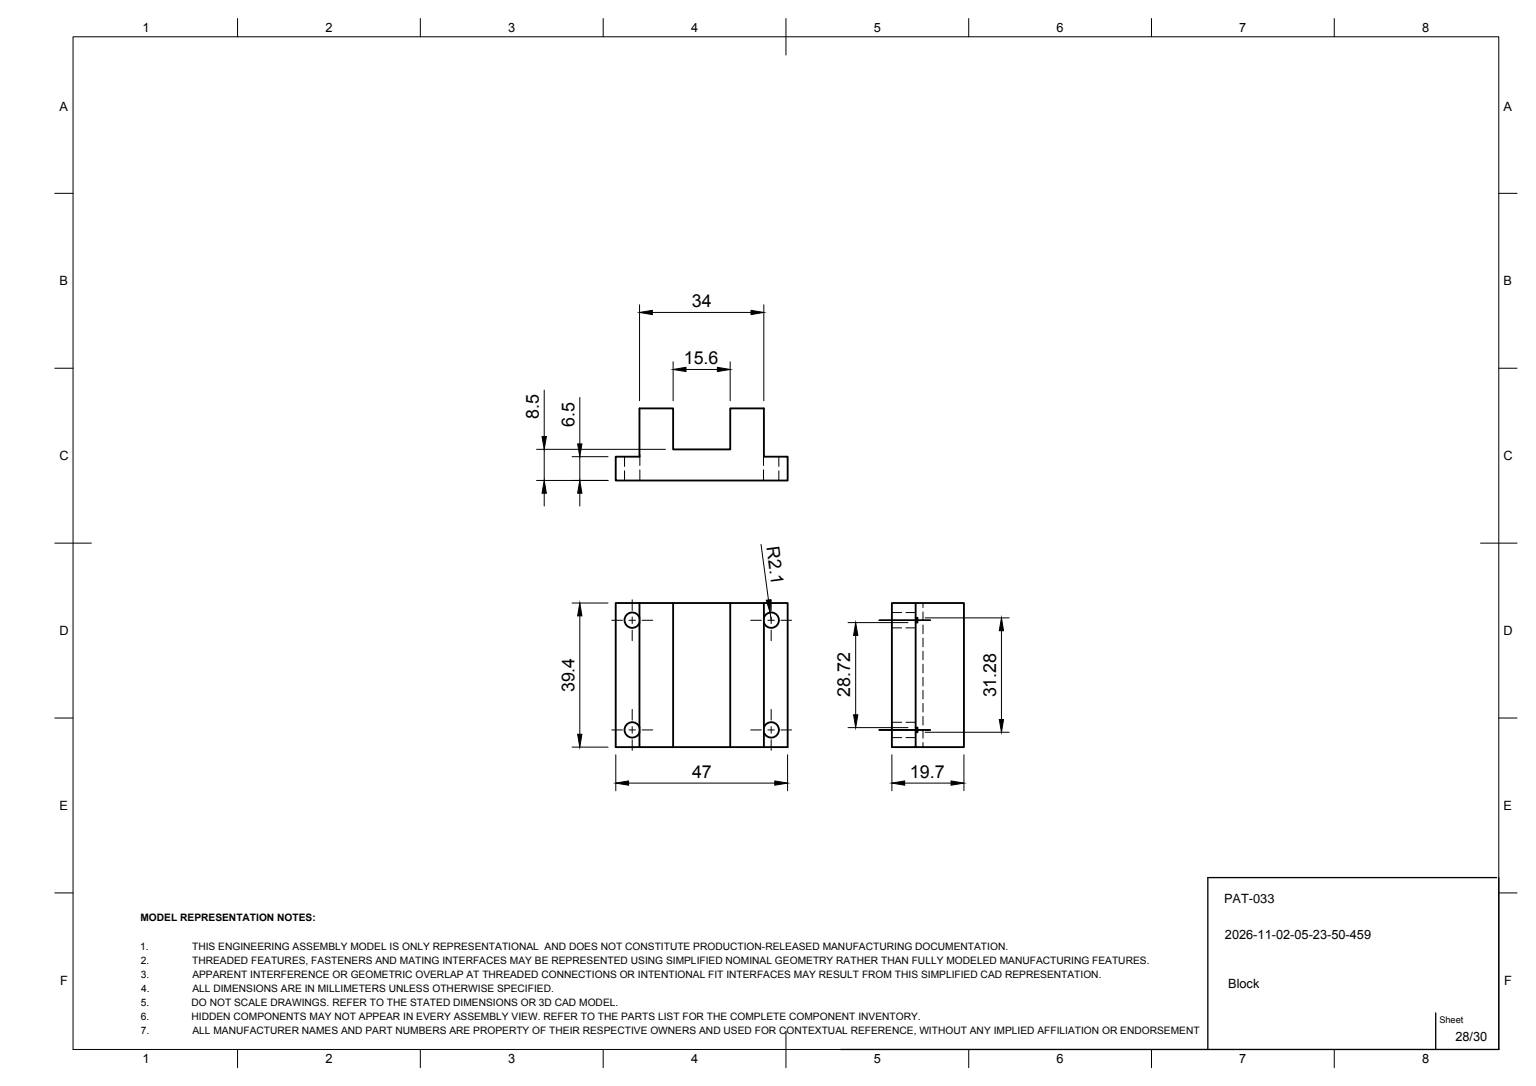
ISO-10303-21;
HEADER;
/* Generated by software containing ST-Developer
 * from STEP Tools, Inc. (www.steptools.com) 
 */

FILE_DESCRIPTION(
/* description */ ('Dual-rail gantry carriage'),
/* implementation_level */ '2;1');

FILE_NAME(
/* name */ 'Block.step',
/* time_stamp */ '2026-10-27T10:49:15-07:00',
/* author */ (''),
/* organization */ (''),
/* preprocessor_version */ 'ST-DEVELOPER v20.2',
/* originating_system */ 'Autodesk Translation Framework v15.17.0.0',
/* authorisation */ '');

FILE_SCHEMA (('AUTOMOTIVE_DESIGN { 1 0 10303 214 3 1 1 }'));
ENDSEC;

DATA;
#10=MECHANICAL_DESIGN_GEOMETRIC_PRESENTATION_REPRESENTATION('',(#607),#12804);
#545=SHAPE_REPRESENTATION_RELATIONSHIP('SRR','None',#13025,#576);
#576=ADVANCED_BREP_SHAPE_REPRESENTATION('',(#636),#12795);
#607=STYLED_ITEM('',(#13226),#636);
#636=MANIFOLD_SOLID_BREP('Body1',#7387);
#751=FACE_BOUND('',#1843,.T.);
#752=FACE_BOUND('',#1844,.T.);
#753=FACE_BOUND('',#1845,.T.);
#754=FACE_BOUND('',#1846,.T.);
#971=PLANE('',#8200);
#972=PLANE('',#8206);
#973=PLANE('',#8212);
#974=PLANE('',#8218);
#975=PLANE('',#8224);
#976=PLANE('',#8225);
#977=PLANE('',#8226);
#978=PLANE('',#8227);
#979=PLANE('',#8228);
#980=PLANE('',#8229);
#981=PLANE('',#8230);
#982=PLANE('',#8231);
#983=PLANE('',#8232);
#984=PLANE('',#8233);
#985=PLANE('',#8234);
#986=PLANE('',#8235);
#987=PLANE('',#8236);
#988=PLANE('',#8237);
#1331=FACE_OUTER_BOUND('',#1829,.T.);
#1332=FACE_OUTER_BOUND('',#1830,.T.);
#1333=FACE_OUTER_BOUND('',#1831,.T.);
#1334=FACE_OUTER_BOUND('',#1832,.T.);
#1335=FACE_OUTER_BOUND('',#1833,.T.);
#1336=FACE_OUTER_BOUND('',#1834,.T.);
#1337=FACE_OUTER_BOUND('',#1835,.T.);
#1338=FACE_OUTER_BOUND('',#1836,.T.);
#1339=FACE_OUTER_BOUND('',#1837,.T.);
#1340=FACE_OUTER_BOUND('',#1838,.T.);
#1341=FACE_OUTER_BOUND('',#1839,.T.);
#1342=FACE_OUTER_BOUND('',#1840,.T.);
#1343=FACE_OUTER_BOUND('',#1841,.T.);
#1344=FACE_OUTER_BOUND('',#1842,.T.);
#1345=FACE_OUTER_BOUND('',#1847,.T.);
#1346=FACE_OUTER_BOUND('',#1848,.T.);
#1347=FACE_OUTER_BOUND('',#1849,.T.);
#1348=FACE_OUTER_BOUND('',#1850,.T.);
#1349=FACE_OUTER_BOUND('',#1851,.T.);
#1350=FACE_OUTER_BOUND('',#1852,.T.);
#1351=FACE_OUTER_BOUND('',#1853,.T.);
#1352=FACE_OUTER_BOUND('',#1854,.T.);
#1829=EDGE_LOOP('',(#6417,#6418));
#1830=EDGE_LOOP('',(#6419,#6420,#6421,#6422,#6423,#6424,#6425,#6426));
#1831=EDGE_LOOP('',(#6427,#6428));
#1832=EDGE_LOOP('',(#6429,#6430,#6431,#6432,#6433,#6434,#6435,#6436));
#1833=EDGE_LOOP('',(#6437,#6438));
#1834=EDGE_LOOP('',(#6439,#6440,#6441,#6442,#6443,#6444,#6445,#6446));
#1835=EDGE_LOOP('',(#6447,#6448));
#1836=EDGE_LOOP('',(#6449,#6450,#6451,#6452,#6453,#6454,#6455,#6456));
#1837=EDGE_LOOP('',(#6457,#6458,#6459,#6460,#6461,#6462,#6463,#6464,#6465,
#6466,#6467,#6468));
#1838=EDGE_LOOP('',(#6469,#6470,#6471,#6472,#6473,#6474,#6475,#6476,#6477,
#6478,#6479,#6480));
#1839=EDGE_LOOP('',(#6481,#6482,#6483,#6484,#6485,#6486,#6487,#6488,#6489,
#6490,#6491,#6492));
#1840=EDGE_LOOP('',(#6493,#6494,#6495,#6496,#6497,#6498,#6499,#6500,#6501,
#6502));
#1841=EDGE_LOOP('',(#6503,#6504,#6505,#6506));
#1842=EDGE_LOOP('',(#6507,#6508,#6509,#6510));
#1843=EDGE_LOOP('',(#6511));
#1844=EDGE_LOOP('',(#6512));
#1845=EDGE_LOOP('',(#6513));
#1846=EDGE_LOOP('',(#6514));
#1847=EDGE_LOOP('',(#6515,#6516,#6517,#6518));
#1848=EDGE_LOOP('',(#6519,#6520,#6521,#6522,#6523,#6524,#6525,#6526,#6527,
#6528));
#1849=EDGE_LOOP('',(#6529,#6530,#6531,#6532));
#1850=EDGE_LOOP('',(#6533,#6534,#6535,#6536));
#1851=EDGE_LOOP('',(#6537,#6538,#6539,#6540));
#1852=EDGE_LOOP('',(#6541,#6542,#6543,#6544));
#1853=EDGE_LOOP('',(#6545,#6546,#6547,#6548));
#1854=EDGE_LOOP('',(#6549,#6550,#6551,#6552,#6553,#6554,#6555,#6556,#6557,
#6558,#6559,#6560));
#2474=LINE('',#12113,#3183);
#2475=LINE('',#12117,#3184);
#2476=LINE('',#12121,#3185);
#2477=LINE('',#12125,#3186);
#2478=LINE('',#12129,#3187);
#2479=LINE('',#12133,#3188);
#2480=LINE('',#12137,#3189);
#2481=LINE('',#12141,#3190);
#2482=LINE('',#12145,#3191);
#2483=LINE('',#12149,#3192);
#2484=LINE('',#12153,#3193);
#2485=LINE('',#12157,#3194);
#2486=LINE('',#12161,#3195);
#2487=LINE('',#12165,#3196);
#2488=LINE('',#12169,#3197);
#2489=LINE('',#12173,#3198);
#2490=LINE('',#12175,#3199);
#2491=LINE('',#12177,#3200);
#2492=LINE('',#12179,#3201);
#2493=LINE('',#12181,#3202);
#2494=LINE('',#12183,#3203);
#2495=LINE('',#12184,#3204);
#2496=LINE('',#12186,#3205);
#2497=LINE('',#12188,#3206);
#2498=LINE('',#12190,#3207);
#2499=LINE('',#12192,#3208);
#2500=LINE('',#12194,#3209);
#2501=LINE('',#12195,#3210);
#2502=LINE('',#12198,#3211);
#2503=LINE('',#12200,#3212);
#2504=LINE('',#12202,#3213);
#2505=LINE('',#12204,#3214);
#2506=LINE('',#12205,#3215);
#2507=LINE('',#12207,#3216);
#2508=LINE('',#12209,#3217);
#2509=LINE('',#12211,#3218);
#2510=LINE('',#12213,#3219);
#2511=LINE('',#12214,#3220);
#2512=LINE('',#12217,#3221);
#2513=LINE('',#12218,#3222);
#2514=LINE('',#12221,#3223);
#2515=LINE('',#12222,#3224);
#2516=LINE('',#12225,#3225);
#2517=LINE('',#12226,#3226);
#2518=LINE('',#12229,#3227);
#2519=LINE('',#12230,#3228);
#2520=LINE('',#12232,#3229);
#2521=LINE('',#12235,#3230);
#2522=LINE('',#12236,#3231);
#2523=LINE('',#12239,#3232);
#2524=LINE('',#12240,#3233);
#2525=LINE('',#12243,#3234);
#2526=LINE('',#12244,#3235);
#2527=LINE('',#12247,#3236);
#2528=LINE('',#12248,#3237);
#2529=LINE('',#12250,#3238);
#3183=VECTOR('',#9933,1.);
#3184=VECTOR('',#9938,1.);
#3185=VECTOR('',#9941,0.21);
#3186=VECTOR('',#9946,1.);
#3187=VECTOR('',#9949,1.);
#3188=VECTOR('',#9954,1.);
#3189=VECTOR('',#9957,0.21);
#3190=VECTOR('',#9962,1.);
#3191=VECTOR('',#9965,1.);
#3192=VECTOR('',#9970,1.);
#3193=VECTOR('',#9973,0.21);
#3194=VECTOR('',#9978,1.);
#3195=VECTOR('',#9981,1.);
#3196=VECTOR('',#9986,1.);
#3197=VECTOR('',#9989,0.21);
#3198=VECTOR('',#9994,1.);
#3199=VECTOR('',#9997,1.);
#3200=VECTOR('',#9998,1.);
#3201=VECTOR('',#9999,1.);
#3202=VECTOR('',#10000,1.);
#3203=VECTOR('',#10001,1.);
#3204=VECTOR('',#10002,1.);
#3205=VECTOR('',#10005,1.);
#3206=VECTOR('',#10006,1.);
#3207=VECTOR('',#10007,1.);
#3208=VECTOR('',#10008,1.);
#3209=VECTOR('',#10009,1.);
#3210=VECTOR('',#10010,1.);
#3211=VECTOR('',#10013,1.);
#3212=VECTOR('',#10014,1.);
#3213=VECTOR('',#10015,1.);
#3214=VECTOR('',#10016,1.);
#3215=VECTOR('',#10017,1.);
#3216=VECTOR('',#10018,1.);
#3217=VECTOR('',#10019,1.);
#3218=VECTOR('',#10020,1.);
#3219=VECTOR('',#10021,1.);
#3220=VECTOR('',#10022,1.);
#3221=VECTOR('',#10025,1.);
#3222=VECTOR('',#10026,1.);
#3223=VECTOR('',#10029,1.);
#3224=VECTOR('',#10030,1.);
#3225=VECTOR('',#10033,1.);
#3226=VECTOR('',#10034,1.);
#3227=VECTOR('',#10037,1.);
#3228=VECTOR('',#10038,1.);
#3229=VECTOR('',#10041,1.);
#3230=VECTOR('',#10044,1.);
#3231=VECTOR('',#10045,1.);
#3232=VECTOR('',#10048,1.);
#3233=VECTOR('',#10049,1.);
#3234=VECTOR('',#10052,1.);
#3235=VECTOR('',#10053,1.);
#3236=VECTOR('',#10056,1.);
#3237=VECTOR('',#10057,1.);
#3238=VECTOR('',#10060,1.);
#3513=CIRCLE('',#8201,0.21);
#3514=CIRCLE('',#8203,0.21);
#3515=CIRCLE('',#8204,0.21);
#3516=CIRCLE('',#8205,0.21);
#3517=CIRCLE('',#8207,0.21);
#3518=CIRCLE('',#8209,0.21);
#3519=CIRCLE('',#8210,0.21);
#3520=CIRCLE('',#8211,0.21);
#3521=CIRCLE('',#8213,0.21);
#3522=CIRCLE('',#8215,0.21);
#3523=CIRCLE('',#8216,0.21);
#3524=CIRCLE('',#8217,0.21);
#3525=CIRCLE('',#8219,0.21);
#3526=CIRCLE('',#8221,0.21);
#3527=CIRCLE('',#8222,0.21);
#3528=CIRCLE('',#8223,0.21);
#4003=VERTEX_POINT('',#12111);
#4004=VERTEX_POINT('',#12112);
#4005=VERTEX_POINT('',#12116);
#4006=VERTEX_POINT('',#12118);
#4007=VERTEX_POINT('',#12120);
#4008=VERTEX_POINT('',#12123);
#4009=VERTEX_POINT('',#12127);
#4010=VERTEX_POINT('',#12128);
#4011=VERTEX_POINT('',#12132);
#4012=VERTEX_POINT('',#12134);
#4013=VERTEX_POINT('',#12136);
#4014=VERTEX_POINT('',#12139);
#4015=VERTEX_POINT('',#12143);
#4016=VERTEX_POINT('',#12144);
#4017=VERTEX_POINT('',#12148);
#4018=VERTEX_POINT('',#12150);
#4019=VERTEX_POINT('',#12152);
#4020=VERTEX_POINT('',#12155);
#4021=VERTEX_POINT('',#12159);
#4022=VERTEX_POINT('',#12160);
#4023=VERTEX_POINT('',#12164);
#4024=VERTEX_POINT('',#12166);
#4025=VERTEX_POINT('',#12168);
#4026=VERTEX_POINT('',#12171);
#4027=VERTEX_POINT('',#12176);
#4028=VERTEX_POINT('',#12178);
#4029=VERTEX_POINT('',#12180);
#4030=VERTEX_POINT('',#12182);
#4031=VERTEX_POINT('',#12187);
#4032=VERTEX_POINT('',#12189);
#4033=VERTEX_POINT('',#12191);
#4034=VERTEX_POINT('',#12193);
#4035=VERTEX_POINT('',#12197);
#4036=VERTEX_POINT('',#12199);
#4037=VERTEX_POINT('',#12201);
#4038=VERTEX_POINT('',#12203);
#4039=VERTEX_POINT('',#12206);
#4040=VERTEX_POINT('',#12208);
#4041=VERTEX_POINT('',#12210);
#4042=VERTEX_POINT('',#12212);
#4043=VERTEX_POINT('',#12216);
#4044=VERTEX_POINT('',#12220);
#4045=VERTEX_POINT('',#12224);
#4046=VERTEX_POINT('',#12228);
#4047=VERTEX_POINT('',#12234);
#4048=VERTEX_POINT('',#12238);
#4049=VERTEX_POINT('',#12242);
#4050=VERTEX_POINT('',#12246);
#4831=EDGE_CURVE('',#4003,#4004,#2474,.T.);
#4832=EDGE_CURVE('',#4003,#4004,#3513,.T.);
#4833=EDGE_CURVE('',#4005,#4003,#2475,.T.);
#4834=EDGE_CURVE('',#4006,#4005,#3514,.T.);
#4835=EDGE_CURVE('',#4006,#4007,#2476,.T.);
#4836=EDGE_CURVE('',#4007,#4007,#3515,.T.);
#4837=EDGE_CURVE('',#4008,#4006,#3516,.T.);
#4838=EDGE_CURVE('',#4004,#4008,#2477,.T.);
#4839=EDGE_CURVE('',#4009,#4010,#2478,.T.);
#4840=EDGE_CURVE('',#4009,#4010,#3517,.T.);
#4841=EDGE_CURVE('',#4011,#4009,#2479,.T.);
#4842=EDGE_CURVE('',#4012,#4011,#3518,.T.);
#4843=EDGE_CURVE('',#4012,#4013,#2480,.T.);
#4844=EDGE_CURVE('',#4013,#4013,#3519,.T.);
#4845=EDGE_CURVE('',#4014,#4012,#3520,.T.);
#4846=EDGE_CURVE('',#4010,#4014,#2481,.T.);
#4847=EDGE_CURVE('',#4015,#4016,#2482,.T.);
#4848=EDGE_CURVE('',#4015,#4016,#3521,.T.);
#4849=EDGE_CURVE('',#4017,#4015,#2483,.T.);
#4850=EDGE_CURVE('',#4018,#4017,#3522,.T.);
#4851=EDGE_CURVE('',#4018,#4019,#2484,.T.);
#4852=EDGE_CURVE('',#4019,#4019,#3523,.T.);
#4853=EDGE_CURVE('',#4020,#4018,#3524,.T.);
#4854=EDGE_CURVE('',#4016,#4020,#2485,.T.);
#4855=EDGE_CURVE('',#4021,#4022,#2486,.T.);
#4856=EDGE_CURVE('',#4021,#4022,#3525,.T.);
#4857=EDGE_CURVE('',#4023,#4021,#2487,.T.);
#4858=EDGE_CURVE('',#4024,#4023,#3526,.T.);
#4859=EDGE_CURVE('',#4024,#4025,#2488,.T.);
#4860=EDGE_CURVE('',#4025,#4025,#3527,.T.);
#4861=EDGE_CURVE('',#4026,#4024,#3528,.T.);
#4862=EDGE_CURVE('',#4022,#4026,#2489,.T.);
#4863=EDGE_CURVE('',#4008,#4017,#2490,.T.);
#4864=EDGE_CURVE('',#4020,#4027,#2491,.T.);
#4865=EDGE_CURVE('',#4028,#4027,#2492,.T.);
#4866=EDGE_CURVE('',#4028,#4029,#2493,.T.);
#4867=EDGE_CURVE('',#4030,#4029,#2494,.T.);
#4868=EDGE_CURVE('',#4030,#4005,#2495,.T.);
#4869=EDGE_CURVE('',#4014,#4023,#2496,.T.);
#4870=EDGE_CURVE('',#4026,#4031,#2497,.T.);
#4871=EDGE_CURVE('',#4032,#4031,#2498,.T.);
#4872=EDGE_CURVE('',#4033,#4032,#2499,.T.);
#4873=EDGE_CURVE('',#4034,#4033,#2500,.T.);
#4874=EDGE_CURVE('',#4034,#4011,#2501,.T.);
#4875=EDGE_CURVE('',#4027,#4035,#2502,.T.);
#4876=EDGE_CURVE('',#4035,#4036,#2503,.T.);
#4877=EDGE_CURVE('',#4036,#4037,#2504,.T.);
#4878=EDGE_CURVE('',#4037,#4038,#2505,.T.);
#4879=EDGE_CURVE('',#4038,#4034,#2506,.T.);
#4880=EDGE_CURVE('',#4033,#4039,#2507,.T.);
#4881=EDGE_CURVE('',#4039,#4040,#2508,.T.);
#4882=EDGE_CURVE('',#4040,#4041,#2509,.T.);
#4883=EDGE_CURVE('',#4041,#4042,#2510,.T.);
#4884=EDGE_CURVE('',#4042,#4028,#2511,.T.);
#4885=EDGE_CURVE('',#4043,#4030,#2512,.T.);
#4886=EDGE_CURVE('',#4035,#4043,#2513,.T.);
#4887=EDGE_CURVE('',#4044,#4043,#2514,.T.);
#4888=EDGE_CURVE('',#4036,#4044,#2515,.T.);
#4889=EDGE_CURVE('',#4045,#4044,#2516,.T.);
#4890=EDGE_CURVE('',#4037,#4045,#2517,.T.);
#4891=EDGE_CURVE('',#4046,#4045,#2518,.T.);
#4892=EDGE_CURVE('',#4038,#4046,#2519,.T.);
#4893=EDGE_CURVE('',#4031,#4046,#2520,.T.);
#4894=EDGE_CURVE('',#4047,#4032,#2521,.T.);
#4895=EDGE_CURVE('',#4039,#4047,#2522,.T.);
#4896=EDGE_CURVE('',#4048,#4047,#2523,.T.);
#4897=EDGE_CURVE('',#4040,#4048,#2524,.T.);
#4898=EDGE_CURVE('',#4049,#4048,#2525,.T.);
#4899=EDGE_CURVE('',#4041,#4049,#2526,.T.);
#4900=EDGE_CURVE('',#4050,#4049,#2527,.T.);
#4901=EDGE_CURVE('',#4042,#4050,#2528,.T.);
#4902=EDGE_CURVE('',#4029,#4050,#2529,.T.);
#6417=ORIENTED_EDGE('',*,*,#4831,.F.);
#6418=ORIENTED_EDGE('',*,*,#4832,.T.);
#6419=ORIENTED_EDGE('',*,*,#4833,.F.);
#6420=ORIENTED_EDGE('',*,*,#4834,.F.);
#6421=ORIENTED_EDGE('',*,*,#4835,.T.);
#6422=ORIENTED_EDGE('',*,*,#4836,.F.);
#6423=ORIENTED_EDGE('',*,*,#4835,.F.);
#6424=ORIENTED_EDGE('',*,*,#4837,.F.);
#6425=ORIENTED_EDGE('',*,*,#4838,.F.);
#6426=ORIENTED_EDGE('',*,*,#4832,.F.);
#6427=ORIENTED_EDGE('',*,*,#4839,.F.);
#6428=ORIENTED_EDGE('',*,*,#4840,.T.);
#6429=ORIENTED_EDGE('',*,*,#4841,.F.);
#6430=ORIENTED_EDGE('',*,*,#4842,.F.);
#6431=ORIENTED_EDGE('',*,*,#4843,.T.);
#6432=ORIENTED_EDGE('',*,*,#4844,.F.);
#6433=ORIENTED_EDGE('',*,*,#4843,.F.);
#6434=ORIENTED_EDGE('',*,*,#4845,.F.);
#6435=ORIENTED_EDGE('',*,*,#4846,.F.);
#6436=ORIENTED_EDGE('',*,*,#4840,.F.);
#6437=ORIENTED_EDGE('',*,*,#4847,.F.);
#6438=ORIENTED_EDGE('',*,*,#4848,.T.);
#6439=ORIENTED_EDGE('',*,*,#4849,.F.);
#6440=ORIENTED_EDGE('',*,*,#4850,.F.);
#6441=ORIENTED_EDGE('',*,*,#4851,.T.);
#6442=ORIENTED_EDGE('',*,*,#4852,.F.);
#6443=ORIENTED_EDGE('',*,*,#4851,.F.);
#6444=ORIENTED_EDGE('',*,*,#4853,.F.);
#6445=ORIENTED_EDGE('',*,*,#4854,.F.);
#6446=ORIENTED_EDGE('',*,*,#4848,.F.);
#6447=ORIENTED_EDGE('',*,*,#4855,.F.);
#6448=ORIENTED_EDGE('',*,*,#4856,.T.);
#6449=ORIENTED_EDGE('',*,*,#4857,.F.);
#6450=ORIENTED_EDGE('',*,*,#4858,.F.);
#6451=ORIENTED_EDGE('',*,*,#4859,.T.);
#6452=ORIENTED_EDGE('',*,*,#4860,.F.);
#6453=ORIENTED_EDGE('',*,*,#4859,.F.);
#6454=ORIENTED_EDGE('',*,*,#4861,.F.);
#6455=ORIENTED_EDGE('',*,*,#4862,.F.);
#6456=ORIENTED_EDGE('',*,*,#4856,.F.);
#6457=ORIENTED_EDGE('',*,*,#4833,.T.);
#6458=ORIENTED_EDGE('',*,*,#4831,.T.);
#6459=ORIENTED_EDGE('',*,*,#4838,.T.);
#6460=ORIENTED_EDGE('',*,*,#4863,.T.);
#6461=ORIENTED_EDGE('',*,*,#4849,.T.);
#6462=ORIENTED_EDGE('',*,*,#4847,.T.);
#6463=ORIENTED_EDGE('',*,*,#4854,.T.);
#6464=ORIENTED_EDGE('',*,*,#4864,.T.);
#6465=ORIENTED_EDGE('',*,*,#4865,.F.);
#6466=ORIENTED_EDGE('',*,*,#4866,.T.);
#6467=ORIENTED_EDGE('',*,*,#4867,.F.);
#6468=ORIENTED_EDGE('',*,*,#4868,.T.);
#6469=ORIENTED_EDGE('',*,*,#4841,.T.);
#6470=ORIENTED_EDGE('',*,*,#4839,.T.);
#6471=ORIENTED_EDGE('',*,*,#4846,.T.);
#6472=ORIENTED_EDGE('',*,*,#4869,.T.);
#6473=ORIENTED_EDGE('',*,*,#4857,.T.);
#6474=ORIENTED_EDGE('',*,*,#4855,.T.);
#6475=ORIENTED_EDGE('',*,*,#4862,.T.);
#6476=ORIENTED_EDGE('',*,*,#4870,.T.);
#6477=ORIENTED_EDGE('',*,*,#4871,.F.);
#6478=ORIENTED_EDGE('',*,*,#4872,.F.);
#6479=ORIENTED_EDGE('',*,*,#4873,.F.);
#6480=ORIENTED_EDGE('',*,*,#4874,.T.);
#6481=ORIENTED_EDGE('',*,*,#4865,.T.);
#6482=ORIENTED_EDGE('',*,*,#4875,.T.);
#6483=ORIENTED_EDGE('',*,*,#4876,.T.);
#6484=ORIENTED_EDGE('',*,*,#4877,.T.);
#6485=ORIENTED_EDGE('',*,*,#4878,.T.);
#6486=ORIENTED_EDGE('',*,*,#4879,.T.);
#6487=ORIENTED_EDGE('',*,*,#4873,.T.);
#6488=ORIENTED_EDGE('',*,*,#4880,.T.);
#6489=ORIENTED_EDGE('',*,*,#4881,.T.);
#6490=ORIENTED_EDGE('',*,*,#4882,.T.);
#6491=ORIENTED_EDGE('',*,*,#4883,.T.);
#6492=ORIENTED_EDGE('',*,*,#4884,.T.);
#6493=ORIENTED_EDGE('',*,*,#4837,.T.);
#6494=ORIENTED_EDGE('',*,*,#4834,.T.);
#6495=ORIENTED_EDGE('',*,*,#4868,.F.);
#6496=ORIENTED_EDGE('',*,*,#4885,.F.);
#6497=ORIENTED_EDGE('',*,*,#4886,.F.);
#6498=ORIENTED_EDGE('',*,*,#4875,.F.);
#6499=ORIENTED_EDGE('',*,*,#4864,.F.);
#6500=ORIENTED_EDGE('',*,*,#4853,.T.);
#6501=ORIENTED_EDGE('',*,*,#4850,.T.);
#6502=ORIENTED_EDGE('',*,*,#4863,.F.);
#6503=ORIENTED_EDGE('',*,*,#4886,.T.);
#6504=ORIENTED_EDGE('',*,*,#4887,.F.);
#6505=ORIENTED_EDGE('',*,*,#4888,.F.);
#6506=ORIENTED_EDGE('',*,*,#4876,.F.);
#6507=ORIENTED_EDGE('',*,*,#4888,.T.);
#6508=ORIENTED_EDGE('',*,*,#4889,.F.);
#6509=ORIENTED_EDGE('',*,*,#4890,.F.);
#6510=ORIENTED_EDGE('',*,*,#4877,.F.);
#6511=ORIENTED_EDGE('',*,*,#4836,.T.);
#6512=ORIENTED_EDGE('',*,*,#4844,.T.);
#6513=ORIENTED_EDGE('',*,*,#4852,.T.);
#6514=ORIENTED_EDGE('',*,*,#4860,.T.);
#6515=ORIENTED_EDGE('',*,*,#4890,.T.);
#6516=ORIENTED_EDGE('',*,*,#4891,.F.);
#6517=ORIENTED_EDGE('',*,*,#4892,.F.);
#6518=ORIENTED_EDGE('',*,*,#4878,.F.);
#6519=ORIENTED_EDGE('',*,*,#4845,.T.);
#6520=ORIENTED_EDGE('',*,*,#4842,.T.);
#6521=ORIENTED_EDGE('',*,*,#4874,.F.);
#6522=ORIENTED_EDGE('',*,*,#4879,.F.);
#6523=ORIENTED_EDGE('',*,*,#4892,.T.);
#6524=ORIENTED_EDGE('',*,*,#4893,.F.);
#6525=ORIENTED_EDGE('',*,*,#4870,.F.);
#6526=ORIENTED_EDGE('',*,*,#4861,.T.);
#6527=ORIENTED_EDGE('',*,*,#4858,.T.);
#6528=ORIENTED_EDGE('',*,*,#4869,.F.);
#6529=ORIENTED_EDGE('',*,*,#4872,.T.);
#6530=ORIENTED_EDGE('',*,*,#4894,.F.);
#6531=ORIENTED_EDGE('',*,*,#4895,.F.);
#6532=ORIENTED_EDGE('',*,*,#4880,.F.);
#6533=ORIENTED_EDGE('',*,*,#4895,.T.);
#6534=ORIENTED_EDGE('',*,*,#4896,.F.);
#6535=ORIENTED_EDGE('',*,*,#4897,.F.);
#6536=ORIENTED_EDGE('',*,*,#4881,.F.);
#6537=ORIENTED_EDGE('',*,*,#4897,.T.);
#6538=ORIENTED_EDGE('',*,*,#4898,.F.);
#6539=ORIENTED_EDGE('',*,*,#4899,.F.);
#6540=ORIENTED_EDGE('',*,*,#4882,.F.);
#6541=ORIENTED_EDGE('',*,*,#4899,.T.);
#6542=ORIENTED_EDGE('',*,*,#4900,.F.);
#6543=ORIENTED_EDGE('',*,*,#4901,.F.);
#6544=ORIENTED_EDGE('',*,*,#4883,.F.);
#6545=ORIENTED_EDGE('',*,*,#4901,.T.);
#6546=ORIENTED_EDGE('',*,*,#4902,.F.);
#6547=ORIENTED_EDGE('',*,*,#4866,.F.);
#6548=ORIENTED_EDGE('',*,*,#4884,.F.);
#6549=ORIENTED_EDGE('',*,*,#4867,.T.);
#6550=ORIENTED_EDGE('',*,*,#4902,.T.);
#6551=ORIENTED_EDGE('',*,*,#4900,.T.);
#6552=ORIENTED_EDGE('',*,*,#4898,.T.);
#6553=ORIENTED_EDGE('',*,*,#4896,.T.);
#6554=ORIENTED_EDGE('',*,*,#4894,.T.);
#6555=ORIENTED_EDGE('',*,*,#4871,.T.);
#6556=ORIENTED_EDGE('',*,*,#4893,.T.);
#6557=ORIENTED_EDGE('',*,*,#4891,.T.);
#6558=ORIENTED_EDGE('',*,*,#4889,.T.);
#6559=ORIENTED_EDGE('',*,*,#4887,.T.);
#6560=ORIENTED_EDGE('',*,*,#4885,.T.);
#6958=CYLINDRICAL_SURFACE('',#8202,0.21);
#6959=CYLINDRICAL_SURFACE('',#8208,0.21);
#6960=CYLINDRICAL_SURFACE('',#8214,0.21);
#6961=CYLINDRICAL_SURFACE('',#8220,0.21);
#7257=ADVANCED_FACE('',(#1331),#971,.T.);
#7258=ADVANCED_FACE('',(#1332),#6958,.F.);
#7259=ADVANCED_FACE('',(#1333),#972,.T.);
#7260=ADVANCED_FACE('',(#1334),#6959,.F.);
#7261=ADVANCED_FACE('',(#1335),#973,.T.);
#7262=ADVANCED_FACE('',(#1336),#6960,.F.);
#7263=ADVANCED_FACE('',(#1337),#974,.T.);
#7264=ADVANCED_FACE('',(#1338),#6961,.F.);
#7265=ADVANCED_FACE('',(#1339),#975,.T.);
#7266=ADVANCED_FACE('',(#1340),#976,.T.);
#7267=ADVANCED_FACE('',(#1341),#977,.T.);
#7268=ADVANCED_FACE('',(#1342),#978,.T.);
#7269=ADVANCED_FACE('',(#1343),#979,.T.);
#7270=ADVANCED_FACE('',(#1344,#751,#752,#753,#754),#980,.T.);
#7271=ADVANCED_FACE('',(#1345),#981,.T.);
#7272=ADVANCED_FACE('',(#1346),#982,.T.);
#7273=ADVANCED_FACE('',(#1347),#983,.T.);
#7274=ADVANCED_FACE('',(#1348),#984,.T.);
#7275=ADVANCED_FACE('',(#1349),#985,.T.);
#7276=ADVANCED_FACE('',(#1350),#986,.T.);
#7277=ADVANCED_FACE('',(#1351),#987,.T.);
#7278=ADVANCED_FACE('',(#1352),#988,.T.);
#7387=CLOSED_SHELL('',(#7257,#7258,#7259,#7260,#7261,#7262,#7263,#7264,
#7265,#7266,#7267,#7268,#7269,#7270,#7271,#7272,#7273,#7274,#7275,#7276,
#7277,#7278));
#8199=AXIS2_PLACEMENT_3D('',#12109,#9929,#9930);
#8200=AXIS2_PLACEMENT_3D('',#12110,#9931,#9932);
#8201=AXIS2_PLACEMENT_3D('',#12114,#9934,#9935);
#8202=AXIS2_PLACEMENT_3D('',#12115,#9936,#9937);
#8203=AXIS2_PLACEMENT_3D('',#12119,#9939,#9940);
#8204=AXIS2_PLACEMENT_3D('',#12122,#9942,#9943);
#8205=AXIS2_PLACEMENT_3D('',#12124,#9944,#9945);
#8206=AXIS2_PLACEMENT_3D('',#12126,#9947,#9948);
#8207=AXIS2_PLACEMENT_3D('',#12130,#9950,#9951);
#8208=AXIS2_PLACEMENT_3D('',#12131,#9952,#9953);
#8209=AXIS2_PLACEMENT_3D('',#12135,#9955,#9956);
#8210=AXIS2_PLACEMENT_3D('',#12138,#9958,#9959);
#8211=AXIS2_PLACEMENT_3D('',#12140,#9960,#9961);
#8212=AXIS2_PLACEMENT_3D('',#12142,#9963,#9964);
#8213=AXIS2_PLACEMENT_3D('',#12146,#9966,#9967);
#8214=AXIS2_PLACEMENT_3D('',#12147,#9968,#9969);
#8215=AXIS2_PLACEMENT_3D('',#12151,#9971,#9972);
#8216=AXIS2_PLACEMENT_3D('',#12154,#9974,#9975);
#8217=AXIS2_PLACEMENT_3D('',#12156,#9976,#9977);
#8218=AXIS2_PLACEMENT_3D('',#12158,#9979,#9980);
#8219=AXIS2_PLACEMENT_3D('',#12162,#9982,#9983);
#8220=AXIS2_PLACEMENT_3D('',#12163,#9984,#9985);
#8221=AXIS2_PLACEMENT_3D('',#12167,#9987,#9988);
#8222=AXIS2_PLACEMENT_3D('',#12170,#9990,#9991);
#8223=AXIS2_PLACEMENT_3D('',#12172,#9992,#9993);
#8224=AXIS2_PLACEMENT_3D('',#12174,#9995,#9996);
#8225=AXIS2_PLACEMENT_3D('',#12185,#10003,#10004);
#8226=AXIS2_PLACEMENT_3D('',#12196,#10011,#10012);
#8227=AXIS2_PLACEMENT_3D('',#12215,#10023,#10024);
#8228=AXIS2_PLACEMENT_3D('',#12219,#10027,#10028);
#8229=AXIS2_PLACEMENT_3D('',#12223,#10031,#10032);
#8230=AXIS2_PLACEMENT_3D('',#12227,#10035,#10036);
#8231=AXIS2_PLACEMENT_3D('',#12231,#10039,#10040);
#8232=AXIS2_PLACEMENT_3D('',#12233,#10042,#10043);
#8233=AXIS2_PLACEMENT_3D('',#12237,#10046,#10047);
#8234=AXIS2_PLACEMENT_3D('',#12241,#10050,#10051);
#8235=AXIS2_PLACEMENT_3D('',#12245,#10054,#10055);
#8236=AXIS2_PLACEMENT_3D('',#12249,#10058,#10059);
#8237=AXIS2_PLACEMENT_3D('',#12251,#10061,#10062);
#9929=DIRECTION('axis',(0.,0.,1.));
#9930=DIRECTION('refdir',(1.,0.,0.));
#9931=DIRECTION('center_axis',(0.,0.,1.));
#9932=DIRECTION('ref_axis',(1.,0.,0.));
#9933=DIRECTION('',(-1.,0.,0.));
#9934=DIRECTION('center_axis',(0.,0.,1.));
#9935=DIRECTION('ref_axis',(1.,0.,0.));
#9936=DIRECTION('center_axis',(0.,0.,1.));
#9937=DIRECTION('ref_axis',(1.,0.,0.));
#9938=DIRECTION('',(0.,0.,-1.));
#9939=DIRECTION('center_axis',(0.,0.,1.));
#9940=DIRECTION('ref_axis',(1.,0.,0.));
#9941=DIRECTION('',(0.,0.,1.));
#9942=DIRECTION('center_axis',(0.,0.,-1.));
#9943=DIRECTION('ref_axis',(1.,0.,0.));
#9944=DIRECTION('center_axis',(0.,0.,1.));
#9945=DIRECTION('ref_axis',(1.,0.,0.));
#9946=DIRECTION('',(0.,0.,1.));
#9947=DIRECTION('center_axis',(0.,0.,1.));
#9948=DIRECTION('ref_axis',(1.,0.,0.));
#9949=DIRECTION('',(1.,0.,0.));
#9950=DIRECTION('center_axis',(0.,0.,1.));
#9951=DIRECTION('ref_axis',(1.,0.,0.));
#9952=DIRECTION('center_axis',(0.,0.,1.));
#9953=DIRECTION('ref_axis',(1.,0.,0.));
#9954=DIRECTION('',(0.,0.,-1.));
#9955=DIRECTION('center_axis',(0.,0.,1.));
#9956=DIRECTION('ref_axis',(1.,0.,0.));
#9957=DIRECTION('',(0.,0.,1.));
#9958=DIRECTION('center_axis',(0.,0.,-1.));
#9959=DIRECTION('ref_axis',(1.,0.,0.));
#9960=DIRECTION('center_axis',(0.,0.,1.));
#9961=DIRECTION('ref_axis',(1.,0.,0.));
#9962=DIRECTION('',(0.,0.,1.));
#9963=DIRECTION('center_axis',(0.,0.,1.));
#9964=DIRECTION('ref_axis',(1.,0.,0.));
#9965=DIRECTION('',(-1.,0.,0.));
#9966=DIRECTION('center_axis',(0.,0.,1.));
#9967=DIRECTION('ref_axis',(1.,0.,0.));
#9968=DIRECTION('center_axis',(0.,0.,1.));
#9969=DIRECTION('ref_axis',(1.,0.,0.));
#9970=DIRECTION('',(0.,0.,-1.));
#9971=DIRECTION('center_axis',(0.,0.,1.));
#9972=DIRECTION('ref_axis',(1.,0.,0.));
#9973=DIRECTION('',(0.,0.,1.));
#9974=DIRECTION('center_axis',(0.,0.,-1.));
#9975=DIRECTION('ref_axis',(1.,0.,0.));
#9976=DIRECTION('center_axis',(0.,0.,1.));
#9977=DIRECTION('ref_axis',(1.,0.,0.));
#9978=DIRECTION('',(0.,0.,1.));
#9979=DIRECTION('center_axis',(0.,0.,1.));
#9980=DIRECTION('ref_axis',(1.,0.,0.));
#9981=DIRECTION('',(1.,0.,0.));
#9982=DIRECTION('center_axis',(0.,0.,1.));
#9983=DIRECTION('ref_axis',(1.,0.,0.));
#9984=DIRECTION('center_axis',(0.,0.,1.));
#9985=DIRECTION('ref_axis',(1.,0.,0.));
#9986=DIRECTION('',(0.,0.,-1.));
#9987=DIRECTION('center_axis',(0.,0.,1.));
#9988=DIRECTION('ref_axis',(1.,0.,0.));
#9989=DIRECTION('',(0.,0.,1.));
#9990=DIRECTION('center_axis',(0.,0.,-1.));
#9991=DIRECTION('ref_axis',(1.,0.,0.));
#9992=DIRECTION('center_axis',(0.,0.,1.));
#9993=DIRECTION('ref_axis',(1.,0.,0.));
#9994=DIRECTION('',(0.,0.,1.));
#9995=DIRECTION('center_axis',(0.,-1.,0.));
#9996=DIRECTION('ref_axis',(0.,0.,-1.));
#9997=DIRECTION('',(-1.,0.,0.));
#9998=DIRECTION('',(-1.,0.,0.));
#9999=DIRECTION('',(0.,0.,1.));
#10000=DIRECTION('',(1.,0.,0.));
#10001=DIRECTION('',(0.,0.,-1.));
#10002=DIRECTION('',(-1.,0.,0.));
#10003=DIRECTION('center_axis',(0.,1.,0.));
#10004=DIRECTION('ref_axis',(0.,0.,1.));
#10005=DIRECTION('',(1.,0.,0.));
#10006=DIRECTION('',(1.,0.,0.));
#10007=DIRECTION('',(0.,0.,1.));
#10008=DIRECTION('',(1.,0.,0.));
#10009=DIRECTION('',(0.,0.,-1.));
#10010=DIRECTION('',(1.,0.,0.));
#10011=DIRECTION('center_axis',(-1.,0.,0.));
#10012=DIRECTION('ref_axis',(0.,0.,1.));
#10013=DIRECTION('',(0.,-1.,0.));
#10014=DIRECTION('',(0.,0.,1.));
#10015=DIRECTION('',(0.,1.,0.));
#10016=DIRECTION('',(0.,0.,-1.));
#10017=DIRECTION('',(0.,-1.,0.));
#10018=DIRECTION('',(0.,-1.,0.));
#10019=DIRECTION('',(0.,0.,1.));
#10020=DIRECTION('',(0.,-1.,0.));
#10021=DIRECTION('',(0.,0.,-1.));
#10022=DIRECTION('',(0.,-1.,0.));
#10023=DIRECTION('center_axis',(0.,0.,-1.));
#10024=DIRECTION('ref_axis',(0.,1.,0.));
#10025=DIRECTION('',(0.,1.,0.));
#10026=DIRECTION('',(1.,0.,0.));
#10027=DIRECTION('center_axis',(0.,-1.,0.));
#10028=DIRECTION('ref_axis',(0.,0.,-1.));
#10029=DIRECTION('',(0.,0.,-1.));
#10030=DIRECTION('',(1.,0.,0.));
#10031=DIRECTION('center_axis',(0.,0.,1.));
#10032=DIRECTION('ref_axis',(0.,-1.,0.));
#10033=DIRECTION('',(0.,-1.,0.));
#10034=DIRECTION('',(1.,0.,0.));
#10035=DIRECTION('center_axis',(0.,1.,0.));
#10036=DIRECTION('ref_axis',(0.,0.,1.));
#10037=DIRECTION('',(0.,0.,1.));
#10038=DIRECTION('',(1.,0.,0.));
#10039=DIRECTION('center_axis',(0.,0.,-1.));
#10040=DIRECTION('ref_axis',(0.,1.,0.));
#10041=DIRECTION('',(0.,1.,0.));
#10042=DIRECTION('center_axis',(0.,0.,-1.));
#10043=DIRECTION('ref_axis',(0.,1.,0.));
#10044=DIRECTION('',(0.,1.,0.));
#10045=DIRECTION('',(1.,0.,0.));
#10046=DIRECTION('center_axis',(0.,-1.,0.));
#10047=DIRECTION('ref_axis',(0.,0.,-1.));
#10048=DIRECTION('',(0.,0.,-1.));
#10049=DIRECTION('',(1.,0.,0.));
#10050=DIRECTION('center_axis',(0.,0.,-1.));
#10051=DIRECTION('ref_axis',(0.,1.,0.));
#10052=DIRECTION('',(0.,1.,0.));
#10053=DIRECTION('',(1.,0.,0.));
#10054=DIRECTION('center_axis',(0.,1.,0.));
#10055=DIRECTION('ref_axis',(0.,0.,1.));
#10056=DIRECTION('',(0.,0.,1.));
#10057=DIRECTION('',(1.,0.,0.));
#10058=DIRECTION('center_axis',(0.,0.,-1.));
#10059=DIRECTION('ref_axis',(0.,1.,0.));
#10060=DIRECTION('',(0.,1.,0.));
#10061=DIRECTION('center_axis',(1.,0.,0.));
#10062=DIRECTION('ref_axis',(0.,0.,-1.));
#12109=CARTESIAN_POINT('',(0.,0.,0.));
#12110=CARTESIAN_POINT('Origin',(1.5,-1.9,1.7));
#12111=CARTESIAN_POINT('',(1.56403124237433,-1.7,1.7));
#12112=CARTESIAN_POINT('',(1.43596875762567,-1.7,1.7));
#12113=CARTESIAN_POINT('',(0.75,-1.7,1.7));
#12114=CARTESIAN_POINT('Origin',(1.5,-1.9,1.7));
#12115=CARTESIAN_POINT('Origin',(1.5,-1.9,1.7));
#12116=CARTESIAN_POINT('',(1.56403124237433,-1.7,1.75));
#12117=CARTESIAN_POINT('',(1.56403124237433,-1.7,1.7));
#12118=CARTESIAN_POINT('',(1.29,-1.9,1.75));
#12119=CARTESIAN_POINT('Origin',(1.5,-1.9,1.75));
#12120=CARTESIAN_POINT('',(1.29,-1.9,2.4));
#12121=CARTESIAN_POINT('',(1.29,-1.9,1.7));
#12122=CARTESIAN_POINT('Origin',(1.5,-1.9,2.4));
#12123=CARTESIAN_POINT('',(1.43596875762567,-1.7,1.75));
#12124=CARTESIAN_POINT('Origin',(1.5,-1.9,1.75));
#12125=CARTESIAN_POINT('',(1.43596875762567,-1.7,1.7));
#12126=CARTESIAN_POINT('Origin',(-1.5,1.9,1.7));
#12127=CARTESIAN_POINT('',(-1.56403124237433,1.7,1.7));
#12128=CARTESIAN_POINT('',(-1.43596875762567,1.7,1.7));
#12129=CARTESIAN_POINT('',(-0.75,1.7,1.7));
#12130=CARTESIAN_POINT('Origin',(-1.5,1.9,1.7));
#12131=CARTESIAN_POINT('Origin',(-1.5,1.9,1.7));
#12132=CARTESIAN_POINT('',(-1.56403124237433,1.7,1.75));
#12133=CARTESIAN_POINT('',(-1.56403124237433,1.7,1.7));
#12134=CARTESIAN_POINT('',(-1.71,1.9,1.75));
#12135=CARTESIAN_POINT('Origin',(-1.5,1.9,1.75));
#12136=CARTESIAN_POINT('',(-1.71,1.9,2.4));
#12137=CARTESIAN_POINT('',(-1.71,1.9,1.7));
#12138=CARTESIAN_POINT('Origin',(-1.5,1.9,2.4));
#12139=CARTESIAN_POINT('',(-1.43596875762567,1.7,1.75));
#12140=CARTESIAN_POINT('Origin',(-1.5,1.9,1.75));
#12141=CARTESIAN_POINT('',(-1.43596875762567,1.7,1.7));
#12142=CARTESIAN_POINT('Origin',(-1.5,-1.9,1.7));
#12143=CARTESIAN_POINT('',(-1.43596875762567,-1.7,1.7));
#12144=CARTESIAN_POINT('',(-1.56403124237433,-1.7,1.7));
#12145=CARTESIAN_POINT('',(-0.75,-1.7,1.7));
#12146=CARTESIAN_POINT('Origin',(-1.5,-1.9,1.7));
#12147=CARTESIAN_POINT('Origin',(-1.5,-1.9,1.7));
#12148=CARTESIAN_POINT('',(-1.43596875762567,-1.7,1.75));
#12149=CARTESIAN_POINT('',(-1.43596875762567,-1.7,1.7));
#12150=CARTESIAN_POINT('',(-1.71,-1.9,1.75));
#12151=CARTESIAN_POINT('Origin',(-1.5,-1.9,1.75));
#12152=CARTESIAN_POINT('',(-1.71,-1.9,2.4));
#12153=CARTESIAN_POINT('',(-1.71,-1.9,1.7));
#12154=CARTESIAN_POINT('Origin',(-1.5,-1.9,2.4));
#12155=CARTESIAN_POINT('',(-1.56403124237433,-1.7,1.75));
#12156=CARTESIAN_POINT('Origin',(-1.5,-1.9,1.75));
#12157=CARTESIAN_POINT('',(-1.56403124237433,-1.7,1.7));
#12158=CARTESIAN_POINT('Origin',(1.5,1.9,1.7));
#12159=CARTESIAN_POINT('',(1.43596875762567,1.7,1.7));
#12160=CARTESIAN_POINT('',(1.56403124237433,1.7,1.7));
#12161=CARTESIAN_POINT('',(0.75,1.7,1.7));
#12162=CARTESIAN_POINT('Origin',(1.5,1.9,1.7));
#12163=CARTESIAN_POINT('Origin',(1.5,1.9,1.7));
#12164=CARTESIAN_POINT('',(1.43596875762567,1.7,1.75));
#12165=CARTESIAN_POINT('',(1.43596875762567,1.7,1.7));
#12166=CARTESIAN_POINT('',(1.29,1.9,1.75));
#12167=CARTESIAN_POINT('Origin',(1.5,1.9,1.75));
#12168=CARTESIAN_POINT('',(1.29,1.9,2.4));
#12169=CARTESIAN_POINT('',(1.29,1.9,1.7));
#12170=CARTESIAN_POINT('Origin',(1.5,1.9,2.4));
#12171=CARTESIAN_POINT('',(1.56403124237433,1.7,1.75));
#12172=CARTESIAN_POINT('Origin',(1.5,1.9,1.75));
#12173=CARTESIAN_POINT('',(1.56403124237433,1.7,1.7));
#12174=CARTESIAN_POINT('Origin',(0.,-1.7,1.75));
#12175=CARTESIAN_POINT('',(0.,-1.7,1.75));
#12176=CARTESIAN_POINT('',(-1.97,-1.7,1.75));
#12177=CARTESIAN_POINT('',(0.,-1.7,1.75));
#12178=CARTESIAN_POINT('',(-1.97,-1.7,0.43));
#12179=CARTESIAN_POINT('',(-1.97,-1.7,1.75));
#12180=CARTESIAN_POINT('',(1.97,-1.7,0.43));
#12181=CARTESIAN_POINT('',(0.,-1.7,0.43));
#12182=CARTESIAN_POINT('',(1.97,-1.7,1.75));
#12183=CARTESIAN_POINT('',(1.97,-1.7,1.75));
#12184=CARTESIAN_POINT('',(0.,-1.7,1.75));
#12185=CARTESIAN_POINT('Origin',(0.,1.7,0.43));
#12186=CARTESIAN_POINT('',(0.,1.7,1.75));
#12187=CARTESIAN_POINT('',(1.97,1.7,1.75));
#12188=CARTESIAN_POINT('',(0.,1.7,1.75));
#12189=CARTESIAN_POINT('',(1.97,1.7,0.43));
#12190=CARTESIAN_POINT('',(1.97,1.7,0.43));
#12191=CARTESIAN_POINT('',(-1.97,1.7,0.43));
#12192=CARTESIAN_POINT('',(0.,1.7,0.43));
#12193=CARTESIAN_POINT('',(-1.97,1.7,1.75));
#12194=CARTESIAN_POINT('',(-1.97,1.7,0.43));
#12195=CARTESIAN_POINT('',(0.,1.7,1.75));
#12196=CARTESIAN_POINT('Origin',(-1.97,0.,1.415));
#12197=CARTESIAN_POINT('',(-1.97,-2.35,1.75));
#12198=CARTESIAN_POINT('',(-1.97,-2.35,1.75));
#12199=CARTESIAN_POINT('',(-1.97,-2.35,2.4));
#12200=CARTESIAN_POINT('',(-1.97,-2.35,2.4));
#12201=CARTESIAN_POINT('',(-1.97,2.35,2.4));
#12202=CARTESIAN_POINT('',(-1.97,2.35,2.4));
#12203=CARTESIAN_POINT('',(-1.97,2.35,1.75));
#12204=CARTESIAN_POINT('',(-1.97,2.35,1.75));
#12205=CARTESIAN_POINT('',(-1.97,1.7,1.75));
#12206=CARTESIAN_POINT('',(-1.97,0.78,0.43));
#12207=CARTESIAN_POINT('',(-1.97,0.78,0.43));
#12208=CARTESIAN_POINT('',(-1.97,0.78,1.55));
#12209=CARTESIAN_POINT('',(-1.97,0.78,1.55));
#12210=CARTESIAN_POINT('',(-1.97,-0.78,1.55));
#12211=CARTESIAN_POINT('',(-1.97,-0.78,1.55));
#12212=CARTESIAN_POINT('',(-1.97,-0.78,0.43));
#12213=CARTESIAN_POINT('',(-1.97,-0.78,0.43));
#12214=CARTESIAN_POINT('',(-1.97,-1.7,0.43));
#12215=CARTESIAN_POINT('Origin',(0.,-2.35,1.75));
#12216=CARTESIAN_POINT('',(1.97,-2.35,1.75));
#12217=CARTESIAN_POINT('',(1.97,-2.35,1.75));
#12218=CARTESIAN_POINT('',(0.,-2.35,1.75));
#12219=CARTESIAN_POINT('Origin',(0.,-2.35,2.4));
#12220=CARTESIAN_POINT('',(1.97,-2.35,2.4));
#12221=CARTESIAN_POINT('',(1.97,-2.35,2.4));
#12222=CARTESIAN_POINT('',(0.,-2.35,2.4));
#12223=CARTESIAN_POINT('Origin',(0.,2.35,2.4));
#12224=CARTESIAN_POINT('',(1.97,2.35,2.4));
#12225=CARTESIAN_POINT('',(1.97,2.35,2.4));
#12226=CARTESIAN_POINT('',(0.,2.35,2.4));
#12227=CARTESIAN_POINT('Origin',(0.,2.35,1.75));
#12228=CARTESIAN_POINT('',(1.97,2.35,1.75));
#12229=CARTESIAN_POINT('',(1.97,2.35,1.75));
#12230=CARTESIAN_POINT('',(0.,2.35,1.75));
#12231=CARTESIAN_POINT('Origin',(0.,1.7,1.75));
#12232=CARTESIAN_POINT('',(1.97,1.7,1.75));
#12233=CARTESIAN_POINT('Origin',(0.,0.78,0.43));
#12234=CARTESIAN_POINT('',(1.97,0.78,0.43));
#12235=CARTESIAN_POINT('',(1.97,0.78,0.43));
#12236=CARTESIAN_POINT('',(0.,0.78,0.43));
#12237=CARTESIAN_POINT('Origin',(0.,0.78,1.55));
#12238=CARTESIAN_POINT('',(1.97,0.78,1.55));
#12239=CARTESIAN_POINT('',(1.97,0.78,1.55));
#12240=CARTESIAN_POINT('',(0.,0.78,1.55));
#12241=CARTESIAN_POINT('Origin',(0.,-0.78,1.55));
#12242=CARTESIAN_POINT('',(1.97,-0.78,1.55));
#12243=CARTESIAN_POINT('',(1.97,-0.78,1.55));
#12244=CARTESIAN_POINT('',(0.,-0.78,1.55));
#12245=CARTESIAN_POINT('Origin',(0.,-0.78,0.43));
#12246=CARTESIAN_POINT('',(1.97,-0.78,0.43));
#12247=CARTESIAN_POINT('',(1.97,-0.78,0.43));
#12248=CARTESIAN_POINT('',(0.,-0.78,0.43));
#12249=CARTESIAN_POINT('Origin',(0.,-1.7,0.43));
#12250=CARTESIAN_POINT('',(1.97,-1.7,0.43));
#12251=CARTESIAN_POINT('Origin',(1.97,0.,1.415));
#12759=UNCERTAINTY_MEASURE_WITH_UNIT(LENGTH_MEASURE(0.001),#12805,
'DISTANCE_ACCURACY_VALUE',
'Maximum model space distance between geometric entities at asserted c
onnectivities');
#12768=UNCERTAINTY_MEASURE_WITH_UNIT(LENGTH_MEASURE(0.001),#12805,
'DISTANCE_ACCURACY_VALUE',
'Maximum model space distance between geometric entities at asserted c
onnectivities');
#12795=(
GEOMETRIC_REPRESENTATION_CONTEXT(3)
GLOBAL_UNCERTAINTY_ASSIGNED_CONTEXT((#12759))
GLOBAL_UNIT_ASSIGNED_CONTEXT((#12805,#12807,#12808))
REPRESENTATION_CONTEXT('','3D')
);
#12804=(
GEOMETRIC_REPRESENTATION_CONTEXT(3)
GLOBAL_UNCERTAINTY_ASSIGNED_CONTEXT((#12768))
GLOBAL_UNIT_ASSIGNED_CONTEXT((#12805,#12807,#12808))
REPRESENTATION_CONTEXT('','3D')
);
#12805=(
LENGTH_UNIT()
NAMED_UNIT(*)
SI_UNIT(.CENTI.,.METRE.)
);
#12807=(
NAMED_UNIT(*)
PLANE_ANGLE_UNIT()
SI_UNIT($,.RADIAN.)
);
#12808=(
NAMED_UNIT(*)
SI_UNIT($,.STERADIAN.)
SOLID_ANGLE_UNIT()
);
#12835=SHAPE_DEFINITION_REPRESENTATION(#12870,#13025);
#12870=PRODUCT_DEFINITION_SHAPE('',$,#13061);
#13025=SHAPE_REPRESENTATION('',(#8199),#12795);
#13034=PRODUCT_DEFINITION_CONTEXT('part definition',#13141,'design');
#13061=PRODUCT_DEFINITION('Block','Block',#13096,#13034);
#13096=PRODUCT_DEFINITION_FORMATION('',$,#13169);
#13141=APPLICATION_CONTEXT(
'Core Data for Automotive Mechanical Design Process');
#13142=PRODUCT_CONTEXT('part definition',#13141,'mechanical');
#13169=PRODUCT('Block','Block','Block',(#13142));
#13220=COLOUR_RGB('Dark Blue',0.08,0.2,0.34);
#13221=FILL_AREA_STYLE_COLOUR('',#13220);
#13222=FILL_AREA_STYLE('',(#13221));
#13223=SURFACE_STYLE_FILL_AREA(#13222);
#13224=SURFACE_SIDE_STYLE('',(#13223));
#13225=SURFACE_STYLE_USAGE(.BOTH.,#13224);
#13226=PRESENTATION_STYLE_ASSIGNMENT((#13225));
ENDSEC;
END-ISO-10303-21;
